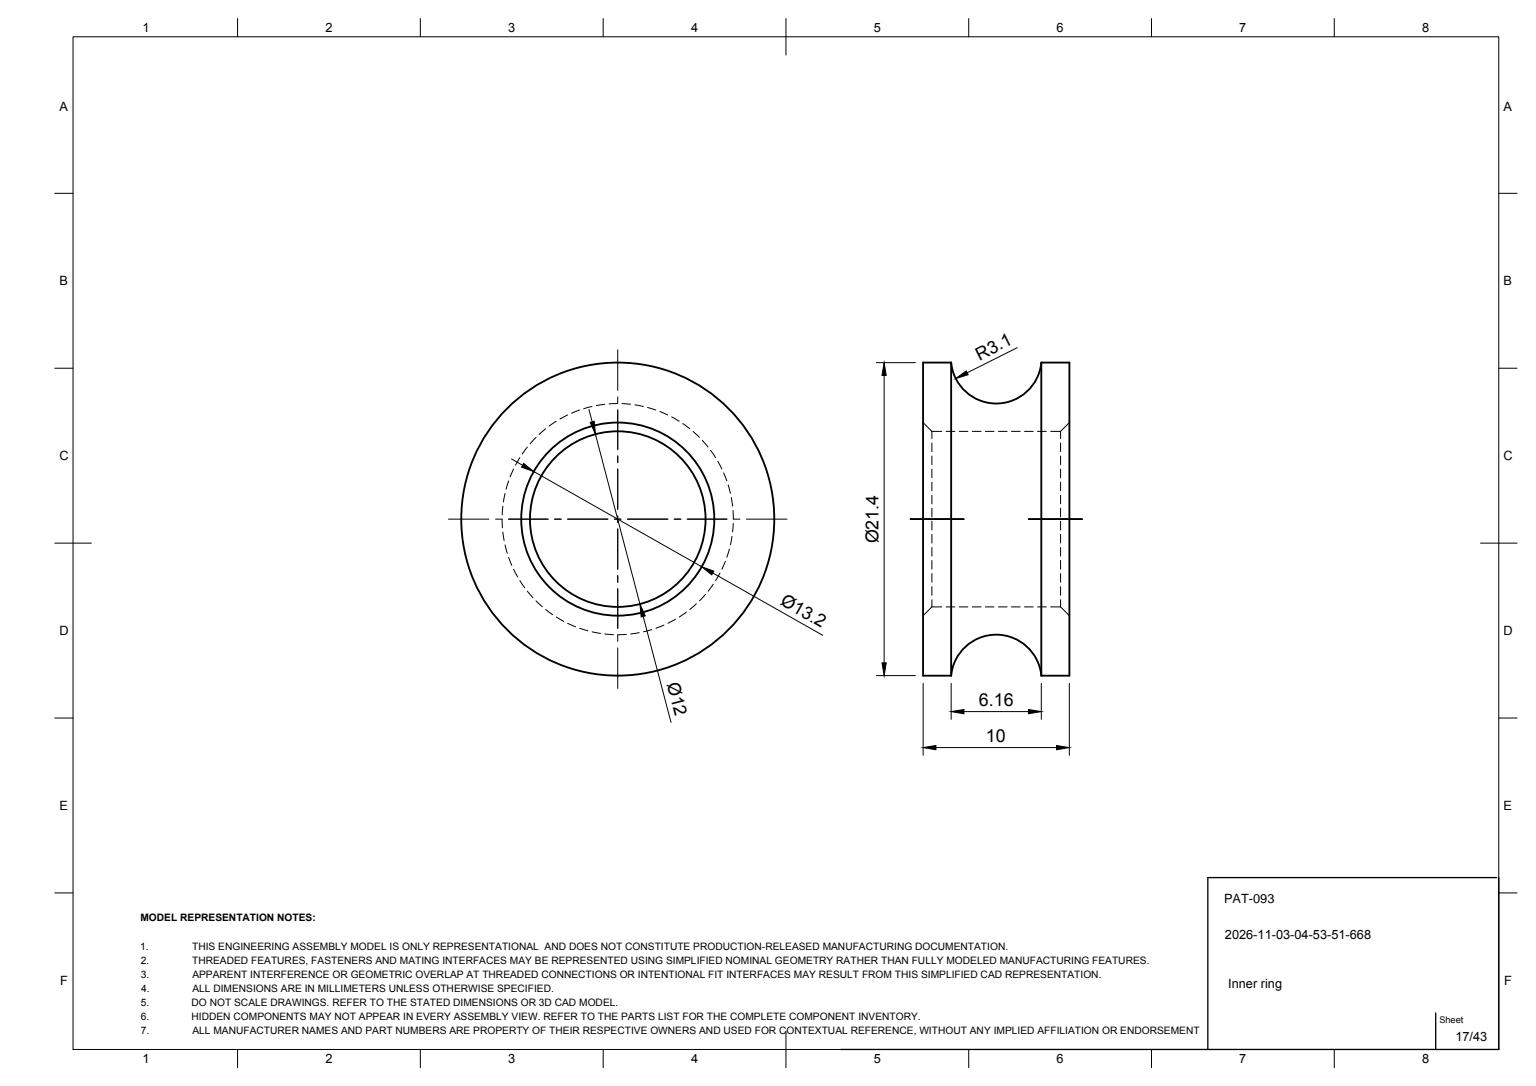
ISO-10303-21;
HEADER;
/* Generated by software containing ST-Developer
 * from STEP Tools, Inc. (www.steptools.com) 
 */

FILE_DESCRIPTION(
/* description */ ('Self-centering screw clamp'),
/* implementation_level */ '2;1');

FILE_NAME(
/* name */ 'Inner ring.step',
/* time_stamp */ '2026-10-28T03:25:31-07:00',
/* author */ (''),
/* organization */ (''),
/* preprocessor_version */ 'ST-DEVELOPER v20.2',
/* originating_system */ 'Autodesk Translation Framework v15.17.0.0',
/* authorisation */ '');

FILE_SCHEMA (('AUTOMOTIVE_DESIGN { 1 0 10303 214 3 1 1 }'));
ENDSEC;

DATA;
#10=MECHANICAL_DESIGN_GEOMETRIC_PRESENTATION_REPRESENTATION('',(#638),#16799);
#481=TOROIDAL_SURFACE('',#9956,1.1,0.309556);
#485=CONICAL_SURFACE('',#9967,0.63,0.785398163397448);
#486=CONICAL_SURFACE('',#9974,0.63,0.785398163397448);
#556=SHAPE_REPRESENTATION_RELATIONSHIP('SRR','None',#17030,#597);
#597=ADVANCED_BREP_SHAPE_REPRESENTATION('',(#686),#16768);
#638=STYLED_ITEM('',(#17326),#686);
#686=MANIFOLD_SOLID_BREP('Body1',#9089);
#842=FACE_BOUND('',#2087,.T.);
#843=FACE_BOUND('',#2090,.T.);
#1106=PLANE('',#9969);
#1107=PLANE('',#9972);
#1454=FACE_OUTER_BOUND('',#2082,.T.);
#1455=FACE_OUTER_BOUND('',#2083,.T.);
#1456=FACE_OUTER_BOUND('',#2084,.T.);
#1457=FACE_OUTER_BOUND('',#2085,.T.);
#1458=FACE_OUTER_BOUND('',#2086,.T.);
#1459=FACE_OUTER_BOUND('',#2088,.T.);
#1460=FACE_OUTER_BOUND('',#2089,.T.);
#1461=FACE_OUTER_BOUND('',#2091,.T.);
#2082=EDGE_LOOP('',(#6993,#6994,#6995,#6996,#6997,#6998));
#2083=EDGE_LOOP('',(#6999,#7000,#7001,#7002,#7003));
#2084=EDGE_LOOP('',(#7004,#7005,#7006,#7007));
#2085=EDGE_LOOP('',(#7008,#7009,#7010,#7011));
#2086=EDGE_LOOP('',(#7012));
#2087=EDGE_LOOP('',(#7013));
#2088=EDGE_LOOP('',(#7014,#7015,#7016,#7017,#7018));
#2089=EDGE_LOOP('',(#7019));
#2090=EDGE_LOOP('',(#7020));
#2091=EDGE_LOOP('',(#7021,#7022,#7023,#7024));
#2826=LINE('',#14695,#3399);
#2827=LINE('',#14701,#3400);
#2828=LINE('',#14705,#3401);
#2829=LINE('',#14711,#3402);
#2830=LINE('',#14716,#3403);
#3399=VECTOR('',#11773,1.070235);
#3400=VECTOR('',#11780,0.6);
#3401=VECTOR('',#11785,0.63);
#3402=VECTOR('',#11794,1.070235);
#3403=VECTOR('',#11801,0.63);
#3903=CIRCLE('',#9957,1.070235);
#3904=CIRCLE('',#9958,1.070235);
#3905=CIRCLE('',#9959,0.309556);
#3906=CIRCLE('',#9960,1.070235);
#3907=CIRCLE('',#9961,1.070235);
#3908=CIRCLE('',#9963,1.070235);
#3909=CIRCLE('',#9965,0.6);
#3910=CIRCLE('',#9966,0.6);
#3911=CIRCLE('',#9968,0.66);
#3912=CIRCLE('',#9971,1.070235);
#3913=CIRCLE('',#9973,0.66);
#4517=VERTEX_POINT('',#14684);
#4518=VERTEX_POINT('',#14685);
#4519=VERTEX_POINT('',#14688);
#4520=VERTEX_POINT('',#14690);
#4521=VERTEX_POINT('',#14694);
#4522=VERTEX_POINT('',#14698);
#4523=VERTEX_POINT('',#14700);
#4524=VERTEX_POINT('',#14704);
#4525=VERTEX_POINT('',#14709);
#4526=VERTEX_POINT('',#14713);
#5421=EDGE_CURVE('',#4517,#4518,#3903,.T.);
#5422=EDGE_CURVE('',#4518,#4517,#3904,.T.);
#5423=EDGE_CURVE('',#4518,#4519,#3905,.T.);
#5424=EDGE_CURVE('',#4520,#4519,#3906,.T.);
#5425=EDGE_CURVE('',#4519,#4520,#3907,.T.);
#5426=EDGE_CURVE('',#4520,#4521,#2826,.T.);
#5427=EDGE_CURVE('',#4521,#4521,#3908,.T.);
#5428=EDGE_CURVE('',#4522,#4522,#3909,.T.);
#5429=EDGE_CURVE('',#4522,#4523,#2827,.T.);
#5430=EDGE_CURVE('',#4523,#4523,#3910,.T.);
#5431=EDGE_CURVE('',#4523,#4524,#2828,.T.);
#5432=EDGE_CURVE('',#4524,#4524,#3911,.T.);
#5433=EDGE_CURVE('',#4525,#4525,#3912,.T.);
#5434=EDGE_CURVE('',#4525,#4517,#2829,.T.);
#5435=EDGE_CURVE('',#4526,#4526,#3913,.T.);
#5436=EDGE_CURVE('',#4526,#4522,#2830,.T.);
#6993=ORIENTED_EDGE('',*,*,#5421,.F.);
#6994=ORIENTED_EDGE('',*,*,#5422,.F.);
#6995=ORIENTED_EDGE('',*,*,#5423,.T.);
#6996=ORIENTED_EDGE('',*,*,#5424,.F.);
#6997=ORIENTED_EDGE('',*,*,#5425,.F.);
#6998=ORIENTED_EDGE('',*,*,#5423,.F.);
#6999=ORIENTED_EDGE('',*,*,#5424,.T.);
#7000=ORIENTED_EDGE('',*,*,#5425,.T.);
#7001=ORIENTED_EDGE('',*,*,#5426,.T.);
#7002=ORIENTED_EDGE('',*,*,#5427,.T.);
#7003=ORIENTED_EDGE('',*,*,#5426,.F.);
#7004=ORIENTED_EDGE('',*,*,#5428,.T.);
#7005=ORIENTED_EDGE('',*,*,#5429,.T.);
#7006=ORIENTED_EDGE('',*,*,#5430,.F.);
#7007=ORIENTED_EDGE('',*,*,#5429,.F.);
#7008=ORIENTED_EDGE('',*,*,#5430,.T.);
#7009=ORIENTED_EDGE('',*,*,#5431,.T.);
#7010=ORIENTED_EDGE('',*,*,#5432,.F.);
#7011=ORIENTED_EDGE('',*,*,#5431,.F.);
#7012=ORIENTED_EDGE('',*,*,#5427,.F.);
#7013=ORIENTED_EDGE('',*,*,#5432,.T.);
#7014=ORIENTED_EDGE('',*,*,#5433,.F.);
#7015=ORIENTED_EDGE('',*,*,#5434,.T.);
#7016=ORIENTED_EDGE('',*,*,#5421,.T.);
#7017=ORIENTED_EDGE('',*,*,#5422,.T.);
#7018=ORIENTED_EDGE('',*,*,#5434,.F.);
#7019=ORIENTED_EDGE('',*,*,#5433,.T.);
#7020=ORIENTED_EDGE('',*,*,#5435,.F.);
#7021=ORIENTED_EDGE('',*,*,#5435,.T.);
#7022=ORIENTED_EDGE('',*,*,#5436,.T.);
#7023=ORIENTED_EDGE('',*,*,#5428,.F.);
#7024=ORIENTED_EDGE('',*,*,#5436,.F.);
#8444=CYLINDRICAL_SURFACE('',#9962,1.070235);
#8445=CYLINDRICAL_SURFACE('',#9964,0.6);
#8446=CYLINDRICAL_SURFACE('',#9970,1.070235);
#8752=ADVANCED_FACE('',(#1454),#481,.F.);
#8753=ADVANCED_FACE('',(#1455),#8444,.T.);
#8754=ADVANCED_FACE('',(#1456),#8445,.F.);
#8755=ADVANCED_FACE('',(#1457),#485,.F.);
#8756=ADVANCED_FACE('',(#1458,#842),#1106,.T.);
#8757=ADVANCED_FACE('',(#1459),#8446,.T.);
#8758=ADVANCED_FACE('',(#1460,#843),#1107,.T.);
#8759=ADVANCED_FACE('',(#1461),#486,.F.);
#9089=CLOSED_SHELL('',(#8752,#8753,#8754,#8755,#8756,#8757,#8758,#8759));
#9955=AXIS2_PLACEMENT_3D('',#14682,#11757,#11758);
#9956=AXIS2_PLACEMENT_3D('',#14683,#11759,#11760);
#9957=AXIS2_PLACEMENT_3D('',#14686,#11761,#11762);
#9958=AXIS2_PLACEMENT_3D('',#14687,#11763,#11764);
#9959=AXIS2_PLACEMENT_3D('',#14689,#11765,#11766);
#9960=AXIS2_PLACEMENT_3D('',#14691,#11767,#11768);
#9961=AXIS2_PLACEMENT_3D('',#14692,#11769,#11770);
#9962=AXIS2_PLACEMENT_3D('',#14693,#11771,#11772);
#9963=AXIS2_PLACEMENT_3D('',#14696,#11774,#11775);
#9964=AXIS2_PLACEMENT_3D('',#14697,#11776,#11777);
#9965=AXIS2_PLACEMENT_3D('',#14699,#11778,#11779);
#9966=AXIS2_PLACEMENT_3D('',#14702,#11781,#11782);
#9967=AXIS2_PLACEMENT_3D('',#14703,#11783,#11784);
#9968=AXIS2_PLACEMENT_3D('',#14706,#11786,#11787);
#9969=AXIS2_PLACEMENT_3D('',#14707,#11788,#11789);
#9970=AXIS2_PLACEMENT_3D('',#14708,#11790,#11791);
#9971=AXIS2_PLACEMENT_3D('',#14710,#11792,#11793);
#9972=AXIS2_PLACEMENT_3D('',#14712,#11795,#11796);
#9973=AXIS2_PLACEMENT_3D('',#14714,#11797,#11798);
#9974=AXIS2_PLACEMENT_3D('',#14715,#11799,#11800);
#11757=DIRECTION('axis',(0.,0.,1.));
#11758=DIRECTION('refdir',(1.,0.,0.));
#11759=DIRECTION('center_axis',(0.,-1.,0.));
#11760=DIRECTION('ref_axis',(0.,0.,-1.));
#11761=DIRECTION('center_axis',(0.,-1.,0.));
#11762=DIRECTION('ref_axis',(1.,0.,0.));
#11763=DIRECTION('center_axis',(0.,-1.,0.));
#11764=DIRECTION('ref_axis',(1.,0.,0.));
#11765=DIRECTION('center_axis',(1.,0.,1.22464679914735E-16));
#11766=DIRECTION('ref_axis',(-1.22464679914735E-16,0.,1.));
#11767=DIRECTION('center_axis',(0.,1.,0.));
#11768=DIRECTION('ref_axis',(1.,0.,0.));
#11769=DIRECTION('center_axis',(0.,1.,0.));
#11770=DIRECTION('ref_axis',(1.,0.,0.));
#11771=DIRECTION('center_axis',(0.,-1.,0.));
#11772=DIRECTION('ref_axis',(1.,0.,0.));
#11773=DIRECTION('',(0.,1.,0.));
#11774=DIRECTION('center_axis',(0.,-1.,0.));
#11775=DIRECTION('ref_axis',(1.,0.,0.));
#11776=DIRECTION('center_axis',(0.,-1.,0.));
#11777=DIRECTION('ref_axis',(1.,0.,0.));
#11778=DIRECTION('center_axis',(0.,-1.,0.));
#11779=DIRECTION('ref_axis',(1.,0.,0.));
#11780=DIRECTION('',(0.,1.,0.));
#11781=DIRECTION('center_axis',(0.,-1.,0.));
#11782=DIRECTION('ref_axis',(1.,0.,0.));
#11783=DIRECTION('center_axis',(0.,1.,0.));
#11784=DIRECTION('ref_axis',(1.,0.,0.));
#11785=DIRECTION('',(-0.707106781186548,0.707106781186547,-8.65956056235493E-17));
#11786=DIRECTION('center_axis',(0.,-1.,0.));
#11787=DIRECTION('ref_axis',(1.,0.,0.));
#11788=DIRECTION('center_axis',(0.,1.,0.));
#11789=DIRECTION('ref_axis',(0.,0.,1.));
#11790=DIRECTION('center_axis',(0.,-1.,0.));
#11791=DIRECTION('ref_axis',(1.,0.,0.));
#11792=DIRECTION('center_axis',(0.,-1.,0.));
#11793=DIRECTION('ref_axis',(1.,0.,0.));
#11794=DIRECTION('',(0.,1.,0.));
#11795=DIRECTION('center_axis',(0.,-1.,0.));
#11796=DIRECTION('ref_axis',(0.,0.,-1.));
#11797=DIRECTION('center_axis',(0.,-1.,0.));
#11798=DIRECTION('ref_axis',(1.,0.,0.));
#11799=DIRECTION('center_axis',(0.,-1.,0.));
#11800=DIRECTION('ref_axis',(1.,0.,0.));
#11801=DIRECTION('',(0.707106781186548,0.707106781186547,8.65956056235493E-17));
#14682=CARTESIAN_POINT('',(0.,0.,0.));
#14683=CARTESIAN_POINT('Origin',(0.,0.,0.));
#14684=CARTESIAN_POINT('',(-1.070235,-0.308121667383195,-1.31065986708547E-16));
#14685=CARTESIAN_POINT('',(-1.31065986708547E-16,-0.308121667383195,1.070235));
#14686=CARTESIAN_POINT('Origin',(0.,-0.308121667383195,0.));
#14687=CARTESIAN_POINT('Origin',(0.,-0.308121667383195,0.));
#14688=CARTESIAN_POINT('',(-1.31065986708547E-16,0.308121667383195,1.070235));
#14689=CARTESIAN_POINT('Origin',(-1.34711147906209E-16,0.,1.1));
#14690=CARTESIAN_POINT('',(-1.070235,0.308121667383195,1.31065986708547E-16));
#14691=CARTESIAN_POINT('Origin',(0.,0.308121667383195,0.));
#14692=CARTESIAN_POINT('Origin',(0.,0.308121667383195,0.));
#14693=CARTESIAN_POINT('Origin',(0.,0.,0.));
#14694=CARTESIAN_POINT('',(-1.070235,0.5,-1.31065986708547E-16));
#14695=CARTESIAN_POINT('',(-1.070235,0.,-1.31065986708547E-16));
#14696=CARTESIAN_POINT('Origin',(0.,0.5,0.));
#14697=CARTESIAN_POINT('Origin',(0.,0.,0.));
#14698=CARTESIAN_POINT('',(-0.6,-0.44,-7.34788079488412E-17));
#14699=CARTESIAN_POINT('Origin',(0.,-0.44,0.));
#14700=CARTESIAN_POINT('',(-0.6,0.44,-7.34788079488412E-17));
#14701=CARTESIAN_POINT('',(-0.6,0.,-7.34788079488412E-17));
#14702=CARTESIAN_POINT('Origin',(0.,0.44,0.));
#14703=CARTESIAN_POINT('Origin',(0.,0.47,0.));
#14704=CARTESIAN_POINT('',(-0.66,0.5,-8.08266887437253E-17));
#14705=CARTESIAN_POINT('',(-0.63,0.47,-7.71527483462832E-17));
#14706=CARTESIAN_POINT('Origin',(0.,0.5,0.));
#14707=CARTESIAN_POINT('Origin',(1.070235,0.5,0.));
#14708=CARTESIAN_POINT('Origin',(0.,0.,0.));
#14709=CARTESIAN_POINT('',(-1.070235,-0.5,-1.31065986708547E-16));
#14710=CARTESIAN_POINT('Origin',(0.,-0.5,0.));
#14711=CARTESIAN_POINT('',(-1.070235,0.,-1.31065986708547E-16));
#14712=CARTESIAN_POINT('Origin',(0.66,-0.5,0.));
#14713=CARTESIAN_POINT('',(-0.66,-0.5,-8.08266887437253E-17));
#14714=CARTESIAN_POINT('Origin',(0.,-0.5,0.));
#14715=CARTESIAN_POINT('Origin',(0.,-0.47,0.));
#14716=CARTESIAN_POINT('',(-0.63,-0.47,-7.71527483462832E-17));
#16719=UNCERTAINTY_MEASURE_WITH_UNIT(LENGTH_MEASURE(0.001),#16800,
'DISTANCE_ACCURACY_VALUE',
'Maximum model space distance between geometric entities at asserted c
onnectivities');
#16750=UNCERTAINTY_MEASURE_WITH_UNIT(LENGTH_MEASURE(0.001),#16800,
'DISTANCE_ACCURACY_VALUE',
'Maximum model space distance between geometric entities at asserted c
onnectivities');
#16768=(
GEOMETRIC_REPRESENTATION_CONTEXT(3)
GLOBAL_UNCERTAINTY_ASSIGNED_CONTEXT((#16719))
GLOBAL_UNIT_ASSIGNED_CONTEXT((#16800,#16802,#16803))
REPRESENTATION_CONTEXT('','3D')
);
#16799=(
GEOMETRIC_REPRESENTATION_CONTEXT(3)
GLOBAL_UNCERTAINTY_ASSIGNED_CONTEXT((#16750))
GLOBAL_UNIT_ASSIGNED_CONTEXT((#16800,#16802,#16803))
REPRESENTATION_CONTEXT('','3D')
);
#16800=(
LENGTH_UNIT()
NAMED_UNIT(*)
SI_UNIT(.CENTI.,.METRE.)
);
#16802=(
NAMED_UNIT(*)
PLANE_ANGLE_UNIT()
SI_UNIT($,.RADIAN.)
);
#16803=(
NAMED_UNIT(*)
SI_UNIT($,.STERADIAN.)
SOLID_ANGLE_UNIT()
);
#16821=SHAPE_DEFINITION_REPRESENTATION(#16869,#17030);
#16869=PRODUCT_DEFINITION_SHAPE('',$,#17079);
#17030=SHAPE_REPRESENTATION('',(#9955),#16768);
#17061=PRODUCT_DEFINITION_CONTEXT('part definition',#17207,'design');
#17079=PRODUCT_DEFINITION('Inner ring','Inner ring',#17127,#17061);
#17127=PRODUCT_DEFINITION_FORMATION('',$,#17226);
#17207=APPLICATION_CONTEXT(
'Core Data for Automotive Mechanical Design Process');
#17208=PRODUCT_CONTEXT('part definition',#17207,'mechanical');
#17226=PRODUCT('Inner ring','Inner ring','Inner ring',(#17208));
#17320=COLOUR_RGB('Grey',0.48,0.52,0.57);
#17321=FILL_AREA_STYLE_COLOUR('',#17320);
#17322=FILL_AREA_STYLE('',(#17321));
#17323=SURFACE_STYLE_FILL_AREA(#17322);
#17324=SURFACE_SIDE_STYLE('',(#17323));
#17325=SURFACE_STYLE_USAGE(.BOTH.,#17324);
#17326=PRESENTATION_STYLE_ASSIGNMENT((#17325));
ENDSEC;
END-ISO-10303-21;
